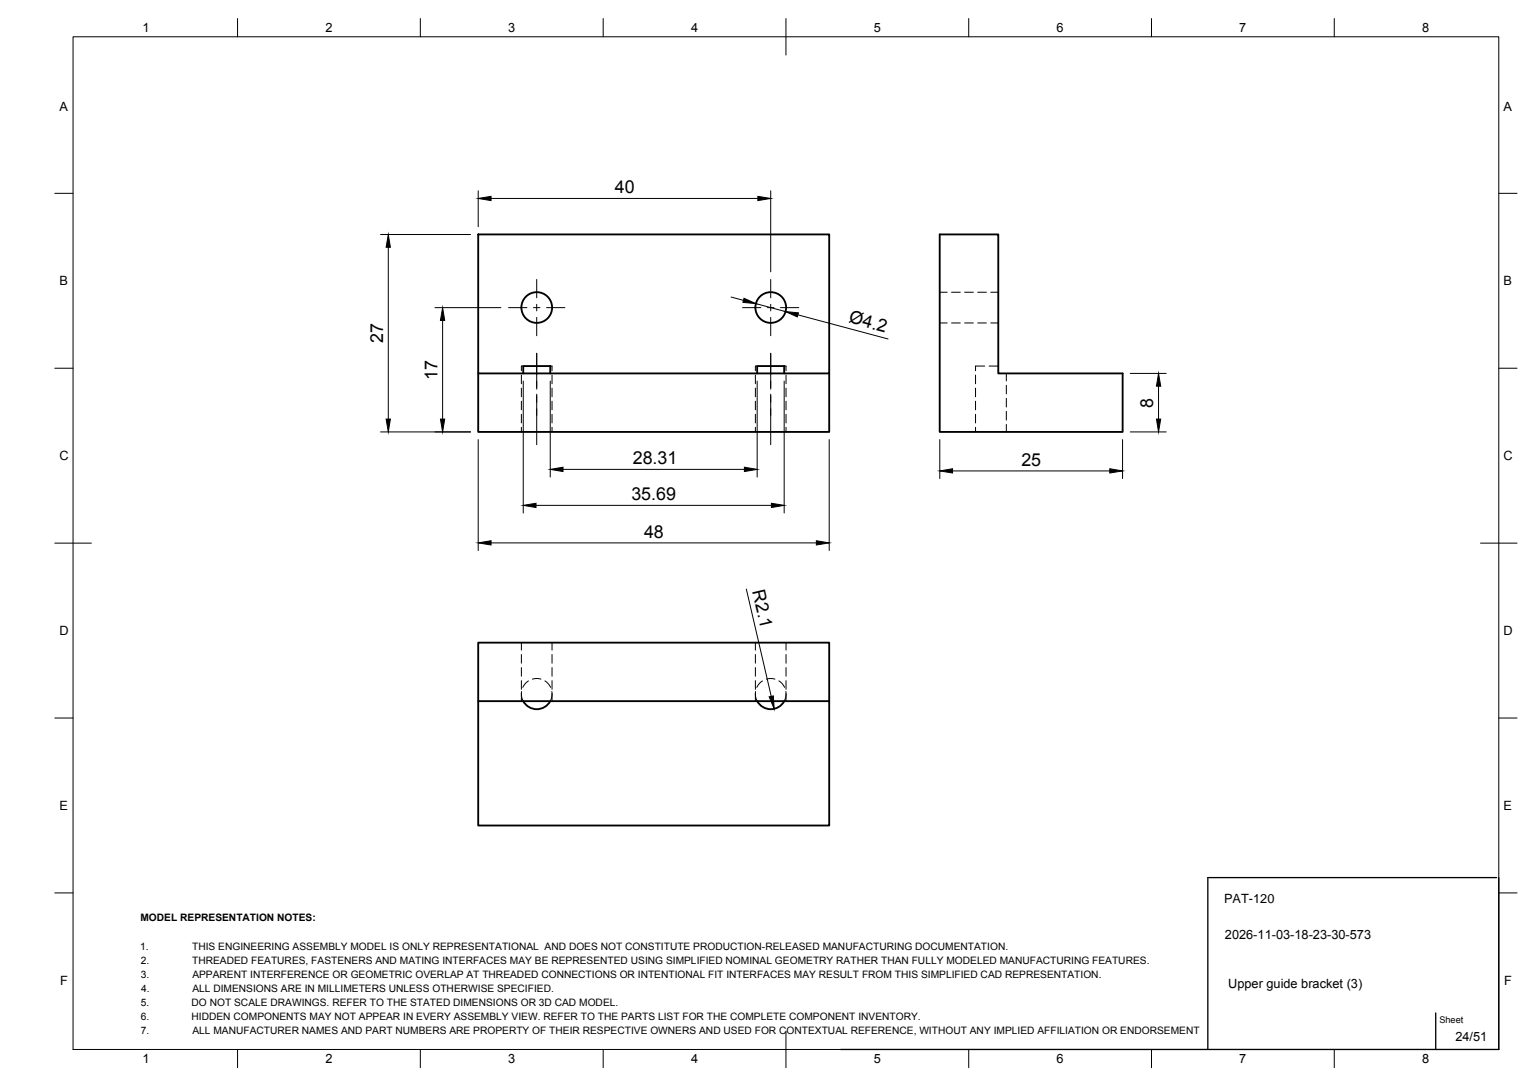
ISO-10303-21;
HEADER;
/* Generated by software containing ST-Developer
 * from STEP Tools, Inc. (www.steptools.com) 
 */

FILE_DESCRIPTION(
/* description */ ('Vibration shaker table dummy'),
/* implementation_level */ '2;1');

FILE_NAME(
/* name */ 'Upper guide bracket (3).step',
/* time_stamp */ '2026-10-27T10:55:14-07:00',
/* author */ (''),
/* organization */ (''),
/* preprocessor_version */ 'ST-DEVELOPER v20.2',
/* originating_system */ 'Autodesk Translation Framework v15.17.0.0',
/* authorisation */ '');

FILE_SCHEMA (('AUTOMOTIVE_DESIGN { 1 0 10303 214 3 1 1 }'));
ENDSEC;

DATA;
#10=MECHANICAL_DESIGN_GEOMETRIC_PRESENTATION_REPRESENTATION('',(#705),#22394);
#613=SHAPE_REPRESENTATION_RELATIONSHIP('SRR','None',#22659,#659);
#659=ADVANCED_BREP_SHAPE_REPRESENTATION('',(#751),#22365);
#705=STYLED_ITEM('',(#22940),#751);
#751=MANIFOLD_SOLID_BREP('Body1',#9223);
#911=FACE_BOUND('',#2186,.T.);
#912=FACE_BOUND('',#2187,.T.);
#913=FACE_BOUND('',#2191,.T.);
#914=FACE_BOUND('',#2192,.T.);
#915=FACE_BOUND('',#2195,.T.);
#916=FACE_BOUND('',#2196,.T.);
#1178=PLANE('',#10175);
#1179=PLANE('',#10181);
#1180=PLANE('',#10182);
#1181=PLANE('',#10183);
#1182=PLANE('',#10184);
#1183=PLANE('',#10185);
#1184=PLANE('',#10186);
#1185=PLANE('',#10187);
#1186=PLANE('',#10188);
#1187=PLANE('',#10189);
#1544=FACE_OUTER_BOUND('',#2178,.T.);
#1545=FACE_OUTER_BOUND('',#2179,.T.);
#1546=FACE_OUTER_BOUND('',#2180,.T.);
#1547=FACE_OUTER_BOUND('',#2181,.T.);
#1548=FACE_OUTER_BOUND('',#2182,.T.);
#1549=FACE_OUTER_BOUND('',#2183,.T.);
#1550=FACE_OUTER_BOUND('',#2184,.T.);
#1551=FACE_OUTER_BOUND('',#2185,.T.);
#1552=FACE_OUTER_BOUND('',#2188,.T.);
#1553=FACE_OUTER_BOUND('',#2189,.T.);
#1554=FACE_OUTER_BOUND('',#2190,.T.);
#1555=FACE_OUTER_BOUND('',#2193,.T.);
#1556=FACE_OUTER_BOUND('',#2194,.T.);
#1557=FACE_OUTER_BOUND('',#2197,.T.);
#2178=EDGE_LOOP('',(#7176,#7177,#7178,#7179));
#2179=EDGE_LOOP('',(#7180,#7181,#7182,#7183));
#2180=EDGE_LOOP('',(#7184,#7185,#7186,#7187,#7188,#7189,#7190,#7191));
#2181=EDGE_LOOP('',(#7192,#7193,#7194));
#2182=EDGE_LOOP('',(#7195,#7196,#7197,#7198,#7199,#7200,#7201,#7202));
#2183=EDGE_LOOP('',(#7203,#7204,#7205));
#2184=EDGE_LOOP('',(#7206,#7207,#7208,#7209,#7210,#7211,#7212,#7213));
#2185=EDGE_LOOP('',(#7214,#7215,#7216,#7217,#7218,#7219,#7220,#7221,#7222,
#7223,#7224,#7225));
#2186=EDGE_LOOP('',(#7226));
#2187=EDGE_LOOP('',(#7227));
#2188=EDGE_LOOP('',(#7228,#7229,#7230,#7231));
#2189=EDGE_LOOP('',(#7232,#7233,#7234,#7235,#7236,#7237));
#2190=EDGE_LOOP('',(#7238,#7239,#7240,#7241));
#2191=EDGE_LOOP('',(#7242));
#2192=EDGE_LOOP('',(#7243));
#2193=EDGE_LOOP('',(#7244,#7245,#7246,#7247,#7248,#7249));
#2194=EDGE_LOOP('',(#7250,#7251,#7252,#7253));
#2195=EDGE_LOOP('',(#7254));
#2196=EDGE_LOOP('',(#7255));
#2197=EDGE_LOOP('',(#7256,#7257,#7258,#7259));
#2902=LINE('',#19336,#3521);
#2903=LINE('',#19342,#3522);
#2904=LINE('',#19348,#3523);
#2905=LINE('',#19352,#3524);
#2906=LINE('',#19356,#3525);
#2907=LINE('',#19359,#3526);
#2908=LINE('',#19364,#3527);
#2909=LINE('',#19368,#3528);
#2910=LINE('',#19372,#3529);
#2911=LINE('',#19375,#3530);
#2912=LINE('',#19377,#3531);
#2913=LINE('',#19379,#3532);
#2914=LINE('',#19381,#3533);
#2915=LINE('',#19383,#3534);
#2916=LINE('',#19385,#3535);
#2917=LINE('',#19386,#3536);
#2918=LINE('',#19389,#3537);
#2919=LINE('',#19391,#3538);
#2920=LINE('',#19392,#3539);
#2921=LINE('',#19396,#3540);
#2922=LINE('',#19397,#3541);
#2923=LINE('',#19398,#3542);
#2924=LINE('',#19402,#3543);
#2925=LINE('',#19403,#3544);
#2926=LINE('',#19404,#3545);
#2927=LINE('',#19408,#3546);
#2928=LINE('',#19409,#3547);
#2929=LINE('',#19410,#3548);
#2930=LINE('',#19412,#3549);
#2931=LINE('',#19413,#3550);
#3521=VECTOR('',#12042,0.21);
#3522=VECTOR('',#12049,0.21);
#3523=VECTOR('',#12056,0.21);
#3524=VECTOR('',#12059,1.);
#3525=VECTOR('',#12062,1.);
#3526=VECTOR('',#12067,1.);
#3527=VECTOR('',#12072,0.21);
#3528=VECTOR('',#12075,1.);
#3529=VECTOR('',#12078,1.);
#3530=VECTOR('',#12083,1.);
#3531=VECTOR('',#12086,1.);
#3532=VECTOR('',#12087,1.);
#3533=VECTOR('',#12088,1.);
#3534=VECTOR('',#12089,1.);
#3535=VECTOR('',#12090,1.);
#3536=VECTOR('',#12091,1.);
#3537=VECTOR('',#12094,1.);
#3538=VECTOR('',#12095,1.);
#3539=VECTOR('',#12096,1.);
#3540=VECTOR('',#12099,1.);
#3541=VECTOR('',#12100,1.);
#3542=VECTOR('',#12101,1.);
#3543=VECTOR('',#12104,1.);
#3544=VECTOR('',#12105,1.);
#3545=VECTOR('',#12106,1.);
#3546=VECTOR('',#12109,1.);
#3547=VECTOR('',#12110,1.);
#3548=VECTOR('',#12111,1.);
#3549=VECTOR('',#12114,1.);
#3550=VECTOR('',#12115,1.);
#4042=CIRCLE('',#10165,0.21);
#4043=CIRCLE('',#10166,0.21);
#4044=CIRCLE('',#10168,0.21);
#4045=CIRCLE('',#10169,0.21);
#4046=CIRCLE('',#10171,0.21);
#4047=CIRCLE('',#10172,0.21);
#4048=CIRCLE('',#10173,0.21);
#4049=CIRCLE('',#10174,0.21);
#4050=CIRCLE('',#10177,0.21);
#4051=CIRCLE('',#10178,0.21);
#4052=CIRCLE('',#10179,0.21);
#4053=CIRCLE('',#10180,0.21);
#4677=VERTEX_POINT('',#19333);
#4678=VERTEX_POINT('',#19335);
#4679=VERTEX_POINT('',#19339);
#4680=VERTEX_POINT('',#19341);
#4681=VERTEX_POINT('',#19345);
#4682=VERTEX_POINT('',#19347);
#4683=VERTEX_POINT('',#19349);
#4684=VERTEX_POINT('',#19351);
#4685=VERTEX_POINT('',#19353);
#4686=VERTEX_POINT('',#19355);
#4687=VERTEX_POINT('',#19361);
#4688=VERTEX_POINT('',#19363);
#4689=VERTEX_POINT('',#19365);
#4690=VERTEX_POINT('',#19367);
#4691=VERTEX_POINT('',#19369);
#4692=VERTEX_POINT('',#19371);
#4693=VERTEX_POINT('',#19378);
#4694=VERTEX_POINT('',#19380);
#4695=VERTEX_POINT('',#19382);
#4696=VERTEX_POINT('',#19384);
#4697=VERTEX_POINT('',#19388);
#4698=VERTEX_POINT('',#19390);
#4699=VERTEX_POINT('',#19394);
#4700=VERTEX_POINT('',#19395);
#4701=VERTEX_POINT('',#19400);
#4702=VERTEX_POINT('',#19401);
#4703=VERTEX_POINT('',#19406);
#4704=VERTEX_POINT('',#19407);
#5581=EDGE_CURVE('',#4677,#4677,#4042,.T.);
#5582=EDGE_CURVE('',#4677,#4678,#2902,.T.);
#5583=EDGE_CURVE('',#4678,#4678,#4043,.T.);
#5584=EDGE_CURVE('',#4679,#4679,#4044,.T.);
#5585=EDGE_CURVE('',#4679,#4680,#2903,.T.);
#5586=EDGE_CURVE('',#4680,#4680,#4045,.T.);
#5587=EDGE_CURVE('',#4681,#4681,#4046,.T.);
#5588=EDGE_CURVE('',#4681,#4682,#2904,.T.);
#5589=EDGE_CURVE('',#4682,#4683,#4047,.T.);
#5590=EDGE_CURVE('',#4684,#4683,#2905,.T.);
#5591=EDGE_CURVE('',#4685,#4684,#4048,.T.);
#5592=EDGE_CURVE('',#4686,#4685,#2906,.T.);
#5593=EDGE_CURVE('',#4686,#4682,#4049,.T.);
#5594=EDGE_CURVE('',#4683,#4686,#2907,.T.);
#5595=EDGE_CURVE('',#4687,#4687,#4050,.T.);
#5596=EDGE_CURVE('',#4687,#4688,#2908,.T.);
#5597=EDGE_CURVE('',#4688,#4689,#4051,.T.);
#5598=EDGE_CURVE('',#4690,#4689,#2909,.T.);
#5599=EDGE_CURVE('',#4691,#4690,#4052,.T.);
#5600=EDGE_CURVE('',#4692,#4691,#2910,.T.);
#5601=EDGE_CURVE('',#4692,#4688,#4053,.T.);
#5602=EDGE_CURVE('',#4689,#4692,#2911,.T.);
#5603=EDGE_CURVE('',#4684,#4691,#2912,.T.);
#5604=EDGE_CURVE('',#4690,#4693,#2913,.T.);
#5605=EDGE_CURVE('',#4694,#4693,#2914,.T.);
#5606=EDGE_CURVE('',#4694,#4695,#2915,.T.);
#5607=EDGE_CURVE('',#4695,#4696,#2916,.T.);
#5608=EDGE_CURVE('',#4696,#4685,#2917,.T.);
#5609=EDGE_CURVE('',#4696,#4697,#2918,.T.);
#5610=EDGE_CURVE('',#4698,#4697,#2919,.T.);
#5611=EDGE_CURVE('',#4693,#4698,#2920,.T.);
#5612=EDGE_CURVE('',#4699,#4700,#2921,.T.);
#5613=EDGE_CURVE('',#4700,#4698,#2922,.T.);
#5614=EDGE_CURVE('',#4697,#4699,#2923,.T.);
#5615=EDGE_CURVE('',#4701,#4702,#2924,.T.);
#5616=EDGE_CURVE('',#4701,#4694,#2925,.T.);
#5617=EDGE_CURVE('',#4702,#4700,#2926,.T.);
#5618=EDGE_CURVE('',#4703,#4704,#2927,.T.);
#5619=EDGE_CURVE('',#4703,#4701,#2928,.T.);
#5620=EDGE_CURVE('',#4704,#4702,#2929,.T.);
#5621=EDGE_CURVE('',#4695,#4703,#2930,.T.);
#5622=EDGE_CURVE('',#4704,#4699,#2931,.T.);
#7176=ORIENTED_EDGE('',*,*,#5581,.F.);
#7177=ORIENTED_EDGE('',*,*,#5582,.T.);
#7178=ORIENTED_EDGE('',*,*,#5583,.F.);
#7179=ORIENTED_EDGE('',*,*,#5582,.F.);
#7180=ORIENTED_EDGE('',*,*,#5584,.F.);
#7181=ORIENTED_EDGE('',*,*,#5585,.T.);
#7182=ORIENTED_EDGE('',*,*,#5586,.F.);
#7183=ORIENTED_EDGE('',*,*,#5585,.F.);
#7184=ORIENTED_EDGE('',*,*,#5587,.F.);
#7185=ORIENTED_EDGE('',*,*,#5588,.T.);
#7186=ORIENTED_EDGE('',*,*,#5589,.T.);
#7187=ORIENTED_EDGE('',*,*,#5590,.F.);
#7188=ORIENTED_EDGE('',*,*,#5591,.F.);
#7189=ORIENTED_EDGE('',*,*,#5592,.F.);
#7190=ORIENTED_EDGE('',*,*,#5593,.T.);
#7191=ORIENTED_EDGE('',*,*,#5588,.F.);
#7192=ORIENTED_EDGE('',*,*,#5594,.F.);
#7193=ORIENTED_EDGE('',*,*,#5589,.F.);
#7194=ORIENTED_EDGE('',*,*,#5593,.F.);
#7195=ORIENTED_EDGE('',*,*,#5595,.F.);
#7196=ORIENTED_EDGE('',*,*,#5596,.T.);
#7197=ORIENTED_EDGE('',*,*,#5597,.T.);
#7198=ORIENTED_EDGE('',*,*,#5598,.F.);
#7199=ORIENTED_EDGE('',*,*,#5599,.F.);
#7200=ORIENTED_EDGE('',*,*,#5600,.F.);
#7201=ORIENTED_EDGE('',*,*,#5601,.T.);
#7202=ORIENTED_EDGE('',*,*,#5596,.F.);
#7203=ORIENTED_EDGE('',*,*,#5602,.F.);
#7204=ORIENTED_EDGE('',*,*,#5597,.F.);
#7205=ORIENTED_EDGE('',*,*,#5601,.F.);
#7206=ORIENTED_EDGE('',*,*,#5591,.T.);
#7207=ORIENTED_EDGE('',*,*,#5603,.T.);
#7208=ORIENTED_EDGE('',*,*,#5599,.T.);
#7209=ORIENTED_EDGE('',*,*,#5604,.T.);
#7210=ORIENTED_EDGE('',*,*,#5605,.F.);
#7211=ORIENTED_EDGE('',*,*,#5606,.T.);
#7212=ORIENTED_EDGE('',*,*,#5607,.T.);
#7213=ORIENTED_EDGE('',*,*,#5608,.T.);
#7214=ORIENTED_EDGE('',*,*,#5592,.T.);
#7215=ORIENTED_EDGE('',*,*,#5608,.F.);
#7216=ORIENTED_EDGE('',*,*,#5609,.T.);
#7217=ORIENTED_EDGE('',*,*,#5610,.F.);
#7218=ORIENTED_EDGE('',*,*,#5611,.F.);
#7219=ORIENTED_EDGE('',*,*,#5604,.F.);
#7220=ORIENTED_EDGE('',*,*,#5598,.T.);
#7221=ORIENTED_EDGE('',*,*,#5602,.T.);
#7222=ORIENTED_EDGE('',*,*,#5600,.T.);
#7223=ORIENTED_EDGE('',*,*,#5603,.F.);
#7224=ORIENTED_EDGE('',*,*,#5590,.T.);
#7225=ORIENTED_EDGE('',*,*,#5594,.T.);
#7226=ORIENTED_EDGE('',*,*,#5581,.T.);
#7227=ORIENTED_EDGE('',*,*,#5584,.T.);
#7228=ORIENTED_EDGE('',*,*,#5612,.T.);
#7229=ORIENTED_EDGE('',*,*,#5613,.T.);
#7230=ORIENTED_EDGE('',*,*,#5610,.T.);
#7231=ORIENTED_EDGE('',*,*,#5614,.T.);
#7232=ORIENTED_EDGE('',*,*,#5615,.F.);
#7233=ORIENTED_EDGE('',*,*,#5616,.T.);
#7234=ORIENTED_EDGE('',*,*,#5605,.T.);
#7235=ORIENTED_EDGE('',*,*,#5611,.T.);
#7236=ORIENTED_EDGE('',*,*,#5613,.F.);
#7237=ORIENTED_EDGE('',*,*,#5617,.F.);
#7238=ORIENTED_EDGE('',*,*,#5618,.F.);
#7239=ORIENTED_EDGE('',*,*,#5619,.T.);
#7240=ORIENTED_EDGE('',*,*,#5615,.T.);
#7241=ORIENTED_EDGE('',*,*,#5620,.F.);
#7242=ORIENTED_EDGE('',*,*,#5587,.T.);
#7243=ORIENTED_EDGE('',*,*,#5595,.T.);
#7244=ORIENTED_EDGE('',*,*,#5607,.F.);
#7245=ORIENTED_EDGE('',*,*,#5621,.T.);
#7246=ORIENTED_EDGE('',*,*,#5618,.T.);
#7247=ORIENTED_EDGE('',*,*,#5622,.T.);
#7248=ORIENTED_EDGE('',*,*,#5614,.F.);
#7249=ORIENTED_EDGE('',*,*,#5609,.F.);
#7250=ORIENTED_EDGE('',*,*,#5622,.F.);
#7251=ORIENTED_EDGE('',*,*,#5620,.T.);
#7252=ORIENTED_EDGE('',*,*,#5617,.T.);
#7253=ORIENTED_EDGE('',*,*,#5612,.F.);
#7254=ORIENTED_EDGE('',*,*,#5583,.T.);
#7255=ORIENTED_EDGE('',*,*,#5586,.T.);
#7256=ORIENTED_EDGE('',*,*,#5621,.F.);
#7257=ORIENTED_EDGE('',*,*,#5606,.F.);
#7258=ORIENTED_EDGE('',*,*,#5616,.F.);
#7259=ORIENTED_EDGE('',*,*,#5619,.F.);
#8588=CYLINDRICAL_SURFACE('',#10164,0.21);
#8589=CYLINDRICAL_SURFACE('',#10167,0.21);
#8590=CYLINDRICAL_SURFACE('',#10170,0.21);
#8591=CYLINDRICAL_SURFACE('',#10176,0.21);
#8909=ADVANCED_FACE('',(#1544),#8588,.F.);
#8910=ADVANCED_FACE('',(#1545),#8589,.F.);
#8911=ADVANCED_FACE('',(#1546),#8590,.F.);
#8912=ADVANCED_FACE('',(#1547),#1178,.F.);
#8913=ADVANCED_FACE('',(#1548),#8591,.F.);
#8914=ADVANCED_FACE('',(#1549),#1179,.F.);
#8915=ADVANCED_FACE('',(#1550),#1180,.T.);
#8916=ADVANCED_FACE('',(#1551,#911,#912),#1181,.T.);
#8917=ADVANCED_FACE('',(#1552),#1182,.T.);
#8918=ADVANCED_FACE('',(#1553),#1183,.T.);
#8919=ADVANCED_FACE('',(#1554,#913,#914),#1184,.T.);
#8920=ADVANCED_FACE('',(#1555),#1185,.T.);
#8921=ADVANCED_FACE('',(#1556,#915,#916),#1186,.T.);
#8922=ADVANCED_FACE('',(#1557),#1187,.F.);
#9223=CLOSED_SHELL('',(#8909,#8910,#8911,#8912,#8913,#8914,#8915,#8916,
#8917,#8918,#8919,#8920,#8921,#8922));
#10163=AXIS2_PLACEMENT_3D('',#19331,#12036,#12037);
#10164=AXIS2_PLACEMENT_3D('',#19332,#12038,#12039);
#10165=AXIS2_PLACEMENT_3D('',#19334,#12040,#12041);
#10166=AXIS2_PLACEMENT_3D('',#19337,#12043,#12044);
#10167=AXIS2_PLACEMENT_3D('',#19338,#12045,#12046);
#10168=AXIS2_PLACEMENT_3D('',#19340,#12047,#12048);
#10169=AXIS2_PLACEMENT_3D('',#19343,#12050,#12051);
#10170=AXIS2_PLACEMENT_3D('',#19344,#12052,#12053);
#10171=AXIS2_PLACEMENT_3D('',#19346,#12054,#12055);
#10172=AXIS2_PLACEMENT_3D('',#19350,#12057,#12058);
#10173=AXIS2_PLACEMENT_3D('',#19354,#12060,#12061);
#10174=AXIS2_PLACEMENT_3D('',#19357,#12063,#12064);
#10175=AXIS2_PLACEMENT_3D('',#19358,#12065,#12066);
#10176=AXIS2_PLACEMENT_3D('',#19360,#12068,#12069);
#10177=AXIS2_PLACEMENT_3D('',#19362,#12070,#12071);
#10178=AXIS2_PLACEMENT_3D('',#19366,#12073,#12074);
#10179=AXIS2_PLACEMENT_3D('',#19370,#12076,#12077);
#10180=AXIS2_PLACEMENT_3D('',#19373,#12079,#12080);
#10181=AXIS2_PLACEMENT_3D('',#19374,#12081,#12082);
#10182=AXIS2_PLACEMENT_3D('',#19376,#12084,#12085);
#10183=AXIS2_PLACEMENT_3D('',#19387,#12092,#12093);
#10184=AXIS2_PLACEMENT_3D('',#19393,#12097,#12098);
#10185=AXIS2_PLACEMENT_3D('',#19399,#12102,#12103);
#10186=AXIS2_PLACEMENT_3D('',#19405,#12107,#12108);
#10187=AXIS2_PLACEMENT_3D('',#19411,#12112,#12113);
#10188=AXIS2_PLACEMENT_3D('',#19414,#12116,#12117);
#10189=AXIS2_PLACEMENT_3D('',#19415,#12118,#12119);
#12036=DIRECTION('axis',(0.,0.,1.));
#12037=DIRECTION('refdir',(1.,0.,0.));
#12038=DIRECTION('center_axis',(0.,0.,1.));
#12039=DIRECTION('ref_axis',(1.,0.,0.));
#12040=DIRECTION('center_axis',(0.,0.,1.));
#12041=DIRECTION('ref_axis',(1.,0.,0.));
#12042=DIRECTION('',(0.,0.,1.));
#12043=DIRECTION('center_axis',(0.,0.,-1.));
#12044=DIRECTION('ref_axis',(1.,0.,0.));
#12045=DIRECTION('center_axis',(0.,0.,1.));
#12046=DIRECTION('ref_axis',(1.,0.,0.));
#12047=DIRECTION('center_axis',(0.,0.,1.));
#12048=DIRECTION('ref_axis',(1.,0.,0.));
#12049=DIRECTION('',(0.,0.,1.));
#12050=DIRECTION('center_axis',(0.,0.,-1.));
#12051=DIRECTION('ref_axis',(1.,0.,0.));
#12052=DIRECTION('center_axis',(0.,1.,0.));
#12053=DIRECTION('ref_axis',(1.,0.,0.));
#12054=DIRECTION('center_axis',(0.,1.,0.));
#12055=DIRECTION('ref_axis',(1.,0.,0.));
#12056=DIRECTION('',(0.,1.,0.));
#12057=DIRECTION('center_axis',(0.,1.,0.));
#12058=DIRECTION('ref_axis',(1.,0.,0.));
#12059=DIRECTION('',(0.,1.,0.));
#12060=DIRECTION('center_axis',(0.,-1.,0.));
#12061=DIRECTION('ref_axis',(1.,0.,0.));
#12062=DIRECTION('',(0.,-1.,0.));
#12063=DIRECTION('center_axis',(0.,1.,0.));
#12064=DIRECTION('ref_axis',(1.,0.,0.));
#12065=DIRECTION('center_axis',(0.,1.,0.));
#12066=DIRECTION('ref_axis',(1.,0.,0.));
#12067=DIRECTION('',(-1.,0.,0.));
#12068=DIRECTION('center_axis',(0.,1.,0.));
#12069=DIRECTION('ref_axis',(1.,0.,0.));
#12070=DIRECTION('center_axis',(0.,1.,0.));
#12071=DIRECTION('ref_axis',(1.,0.,0.));
#12072=DIRECTION('',(0.,1.,0.));
#12073=DIRECTION('center_axis',(0.,1.,0.));
#12074=DIRECTION('ref_axis',(1.,0.,0.));
#12075=DIRECTION('',(0.,1.,0.));
#12076=DIRECTION('center_axis',(0.,-1.,0.));
#12077=DIRECTION('ref_axis',(1.,0.,0.));
#12078=DIRECTION('',(0.,-1.,0.));
#12079=DIRECTION('center_axis',(0.,1.,0.));
#12080=DIRECTION('ref_axis',(1.,0.,0.));
#12081=DIRECTION('center_axis',(0.,1.,0.));
#12082=DIRECTION('ref_axis',(1.,0.,0.));
#12083=DIRECTION('',(-1.,0.,0.));
#12084=DIRECTION('center_axis',(0.,1.,0.));
#12085=DIRECTION('ref_axis',(-1.,0.,0.));
#12086=DIRECTION('',(1.,0.,0.));
#12087=DIRECTION('',(1.,0.,0.));
#12088=DIRECTION('',(0.,0.,1.));
#12089=DIRECTION('',(-1.,0.,0.));
#12090=DIRECTION('',(0.,0.,1.));
#12091=DIRECTION('',(1.,0.,0.));
#12092=DIRECTION('center_axis',(0.,0.,-1.));
#12093=DIRECTION('ref_axis',(-1.,0.,0.));
#12094=DIRECTION('',(0.,1.,0.));
#12095=DIRECTION('',(-1.,0.,0.));
#12096=DIRECTION('',(0.,1.,0.));
#12097=DIRECTION('center_axis',(0.,1.,0.));
#12098=DIRECTION('ref_axis',(0.,0.,1.));
#12099=DIRECTION('',(1.,0.,0.));
#12100=DIRECTION('',(0.,0.,-1.));
#12101=DIRECTION('',(0.,0.,1.));
#12102=DIRECTION('center_axis',(1.,0.,0.));
#12103=DIRECTION('ref_axis',(0.,1.,0.));
#12104=DIRECTION('',(0.,0.,1.));
#12105=DIRECTION('',(0.,1.,0.));
#12106=DIRECTION('',(0.,1.,0.));
#12107=DIRECTION('center_axis',(0.,-1.,0.));
#12108=DIRECTION('ref_axis',(1.,0.,0.));
#12109=DIRECTION('',(0.,0.,1.));
#12110=DIRECTION('',(1.,0.,0.));
#12111=DIRECTION('',(1.,0.,0.));
#12112=DIRECTION('center_axis',(-1.,0.,0.));
#12113=DIRECTION('ref_axis',(0.,-1.,0.));
#12114=DIRECTION('',(0.,-1.,0.));
#12115=DIRECTION('',(0.,1.,0.));
#12116=DIRECTION('center_axis',(0.,0.,1.));
#12117=DIRECTION('ref_axis',(1.,0.,0.));
#12118=DIRECTION('center_axis',(0.,0.,1.));
#12119=DIRECTION('ref_axis',(1.,0.,0.));
#19331=CARTESIAN_POINT('',(0.,0.,0.));
#19332=CARTESIAN_POINT('Origin',(4.4,8.,29.6));
#19333=CARTESIAN_POINT('',(4.19,8.,29.7));
#19334=CARTESIAN_POINT('Origin',(4.4,8.,29.7));
#19335=CARTESIAN_POINT('',(4.19,8.,30.5));
#19336=CARTESIAN_POINT('',(4.19,8.,29.6));
#19337=CARTESIAN_POINT('Origin',(4.4,8.,30.5));
#19338=CARTESIAN_POINT('Origin',(7.6,8.,29.6));
#19339=CARTESIAN_POINT('',(7.39,8.,29.7));
#19340=CARTESIAN_POINT('Origin',(7.6,8.,29.7));
#19341=CARTESIAN_POINT('',(7.39,8.,30.5));
#19342=CARTESIAN_POINT('',(7.39,8.,29.6));
#19343=CARTESIAN_POINT('Origin',(7.6,8.,30.5));
#19344=CARTESIAN_POINT('Origin',(4.4,6.2,29.8));
#19345=CARTESIAN_POINT('',(4.19,6.3,29.8));
#19346=CARTESIAN_POINT('Origin',(4.4,6.3,29.8));
#19347=CARTESIAN_POINT('',(4.19,7.2,29.8));
#19348=CARTESIAN_POINT('',(4.19,6.2,29.8));
#19349=CARTESIAN_POINT('',(4.58466185312619,7.2,29.7));
#19350=CARTESIAN_POINT('Origin',(4.4,7.2,29.8));
#19351=CARTESIAN_POINT('',(4.5846618531262,7.1,29.7));
#19352=CARTESIAN_POINT('',(4.58466185312619,6.2,29.7));
#19353=CARTESIAN_POINT('',(4.21533814687381,7.1,29.7));
#19354=CARTESIAN_POINT('Origin',(4.4,7.1,29.8));
#19355=CARTESIAN_POINT('',(4.21533814687381,7.2,29.7));
#19356=CARTESIAN_POINT('',(4.21533814687381,6.2,29.7));
#19357=CARTESIAN_POINT('Origin',(4.4,7.2,29.8));
#19358=CARTESIAN_POINT('Origin',(4.4,7.2,29.8));
#19359=CARTESIAN_POINT('',(6.4,7.2,29.7));
#19360=CARTESIAN_POINT('Origin',(7.6,6.2,29.8));
#19361=CARTESIAN_POINT('',(7.39,6.3,29.8));
#19362=CARTESIAN_POINT('Origin',(7.6,6.3,29.8));
#19363=CARTESIAN_POINT('',(7.39,7.2,29.8));
#19364=CARTESIAN_POINT('',(7.39,6.2,29.8));
#19365=CARTESIAN_POINT('',(7.78466185312619,7.2,29.7));
#19366=CARTESIAN_POINT('Origin',(7.6,7.2,29.8));
#19367=CARTESIAN_POINT('',(7.78466185312619,7.1,29.7));
#19368=CARTESIAN_POINT('',(7.78466185312619,6.2,29.7));
#19369=CARTESIAN_POINT('',(7.4153381468738,7.1,29.7));
#19370=CARTESIAN_POINT('Origin',(7.6,7.1,29.8));
#19371=CARTESIAN_POINT('',(7.41533814687381,7.2,29.7));
#19372=CARTESIAN_POINT('',(7.41533814687381,6.2,29.7));
#19373=CARTESIAN_POINT('Origin',(7.6,7.2,29.8));
#19374=CARTESIAN_POINT('Origin',(7.6,7.2,29.8));
#19375=CARTESIAN_POINT('',(8.,7.2,29.7));
#19376=CARTESIAN_POINT('Origin',(8.4,7.1,28.));
#19377=CARTESIAN_POINT('',(8.4,7.1,29.7));
#19378=CARTESIAN_POINT('',(8.4,7.1,29.7));
#19379=CARTESIAN_POINT('',(8.4,7.1,29.7));
#19380=CARTESIAN_POINT('',(8.4,7.1,28.));
#19381=CARTESIAN_POINT('',(8.4,7.1,28.));
#19382=CARTESIAN_POINT('',(3.6,7.1,28.));
#19383=CARTESIAN_POINT('',(8.4,7.1,28.));
#19384=CARTESIAN_POINT('',(3.6,7.1,29.7));
#19385=CARTESIAN_POINT('',(3.6,7.1,28.));
#19386=CARTESIAN_POINT('',(8.4,7.1,29.7));
#19387=CARTESIAN_POINT('Origin',(8.4,6.3,29.7));
#19388=CARTESIAN_POINT('',(3.6,9.,29.7));
#19389=CARTESIAN_POINT('',(3.6,6.3,29.7));
#19390=CARTESIAN_POINT('',(8.4,9.,29.7));
#19391=CARTESIAN_POINT('',(3.6,9.,29.7));
#19392=CARTESIAN_POINT('',(8.4,6.3,29.7));
#19393=CARTESIAN_POINT('Origin',(6.,9.,30.1));
#19394=CARTESIAN_POINT('',(3.6,9.,30.5));
#19395=CARTESIAN_POINT('',(8.4,9.,30.5));
#19396=CARTESIAN_POINT('',(8.4,9.,30.5));
#19397=CARTESIAN_POINT('',(8.4,9.,29.7));
#19398=CARTESIAN_POINT('',(3.6,9.,30.5));
#19399=CARTESIAN_POINT('Origin',(8.4,6.3,28.));
#19400=CARTESIAN_POINT('',(8.4,6.3,28.));
#19401=CARTESIAN_POINT('',(8.4,6.3,30.5));
#19402=CARTESIAN_POINT('',(8.4,6.3,28.));
#19403=CARTESIAN_POINT('',(8.4,6.3,28.));
#19404=CARTESIAN_POINT('',(8.4,6.3,30.5));
#19405=CARTESIAN_POINT('Origin',(3.6,6.3,28.));
#19406=CARTESIAN_POINT('',(3.6,6.3,28.));
#19407=CARTESIAN_POINT('',(3.6,6.3,30.5));
#19408=CARTESIAN_POINT('',(3.6,6.3,28.));
#19409=CARTESIAN_POINT('',(3.6,6.3,28.));
#19410=CARTESIAN_POINT('',(3.6,6.3,30.5));
#19411=CARTESIAN_POINT('Origin',(3.6,7.1,28.));
#19412=CARTESIAN_POINT('',(3.6,7.1,28.));
#19413=CARTESIAN_POINT('',(3.6,6.3,30.5));
#19414=CARTESIAN_POINT('Origin',(6.,6.7,30.5));
#19415=CARTESIAN_POINT('Origin',(6.,6.7,28.));
#22314=UNCERTAINTY_MEASURE_WITH_UNIT(LENGTH_MEASURE(0.001),#22395,
'DISTANCE_ACCURACY_VALUE',
'Maximum model space distance between geometric entities at asserted c
onnectivities');
#22343=UNCERTAINTY_MEASURE_WITH_UNIT(LENGTH_MEASURE(0.001),#22395,
'DISTANCE_ACCURACY_VALUE',
'Maximum model space distance between geometric entities at asserted c
onnectivities');
#22365=(
GEOMETRIC_REPRESENTATION_CONTEXT(3)
GLOBAL_UNCERTAINTY_ASSIGNED_CONTEXT((#22314))
GLOBAL_UNIT_ASSIGNED_CONTEXT((#22395,#22397,#22398))
REPRESENTATION_CONTEXT('','3D')
);
#22394=(
GEOMETRIC_REPRESENTATION_CONTEXT(3)
GLOBAL_UNCERTAINTY_ASSIGNED_CONTEXT((#22343))
GLOBAL_UNIT_ASSIGNED_CONTEXT((#22395,#22397,#22398))
REPRESENTATION_CONTEXT('','3D')
);
#22395=(
LENGTH_UNIT()
NAMED_UNIT(*)
SI_UNIT(.CENTI.,.METRE.)
);
#22397=(
NAMED_UNIT(*)
PLANE_ANGLE_UNIT()
SI_UNIT($,.RADIAN.)
);
#22398=(
NAMED_UNIT(*)
SI_UNIT($,.STERADIAN.)
SOLID_ANGLE_UNIT()
);
#22420=SHAPE_DEFINITION_REPRESENTATION(#22470,#22659);
#22470=PRODUCT_DEFINITION_SHAPE('',$,#22710);
#22659=SHAPE_REPRESENTATION('',(#10163),#22365);
#22688=PRODUCT_DEFINITION_CONTEXT('part definition',#22840,'design');
#22710=PRODUCT_DEFINITION('Upper guide bracket (3)',
'Upper guide bracket (3)',#22760,#22688);
#22760=PRODUCT_DEFINITION_FORMATION('',$,#22863);
#22840=APPLICATION_CONTEXT(
'Core Data for Automotive Mechanical Design Process');
#22841=PRODUCT_CONTEXT('part definition',#22840,'mechanical');
#22863=PRODUCT('Upper guide bracket (3)','Upper guide bracket (3)',
'Upper guide bracket (3)',(#22841));
#22934=COLOUR_RGB('Dark Blue',0.08,0.2,0.34);
#22935=FILL_AREA_STYLE_COLOUR('',#22934);
#22936=FILL_AREA_STYLE('',(#22935));
#22937=SURFACE_STYLE_FILL_AREA(#22936);
#22938=SURFACE_SIDE_STYLE('',(#22937));
#22939=SURFACE_STYLE_USAGE(.BOTH.,#22938);
#22940=PRESENTATION_STYLE_ASSIGNMENT((#22939));
ENDSEC;
END-ISO-10303-21;
